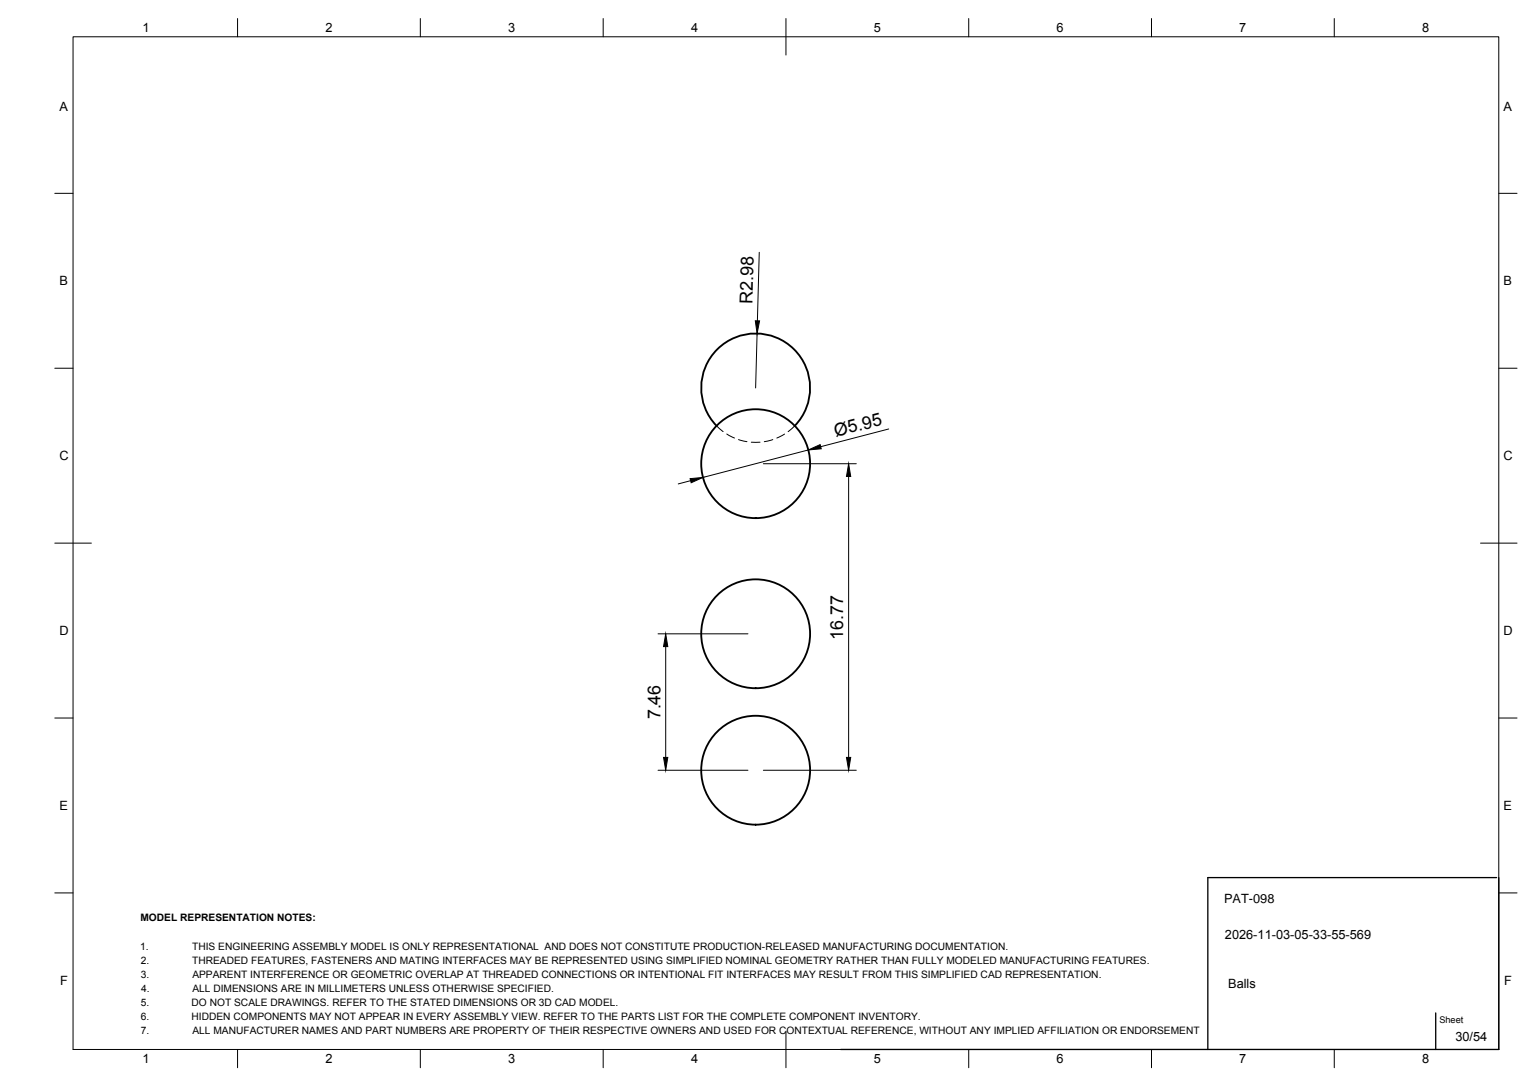
ISO-10303-21;
HEADER;
/* Generated by software containing ST-Developer
 * from STEP Tools, Inc. (www.steptools.com) 
 */

FILE_DESCRIPTION(
/* description */ ('Spring compression tester'),
/* implementation_level */ '2;1');

FILE_NAME(
/* name */ 'Balls.step',
/* time_stamp */ '2026-10-28T03:24:11-07:00',
/* author */ (''),
/* organization */ (''),
/* preprocessor_version */ 'ST-DEVELOPER v20.2',
/* originating_system */ 'Autodesk Translation Framework v15.17.0.0',
/* authorisation */ '');

FILE_SCHEMA (('AUTOMOTIVE_DESIGN { 1 0 10303 214 3 1 1 }'));
ENDSEC;

DATA;
#10=MECHANICAL_DESIGN_GEOMETRIC_PRESENTATION_REPRESENTATION('',(#1129,#1130,#1131,#1132,#1133,#1134,#1135),#43521);
#897=SPHERICAL_SURFACE('',#20034,0.29765);
#898=SPHERICAL_SURFACE('',#20036,0.29765);
#899=SPHERICAL_SURFACE('',#20038,0.29765);
#900=SPHERICAL_SURFACE('',#20040,0.29765);
#901=SPHERICAL_SURFACE('',#20042,0.29765);
#902=SPHERICAL_SURFACE('',#20044,0.29765);
#903=SPHERICAL_SURFACE('',#20046,0.29765);
#1009=SHAPE_REPRESENTATION_RELATIONSHIP('SRR','None',#43822,#1069);
#1069=ADVANCED_BREP_SHAPE_REPRESENTATION('',(#1203,#1204,#1205,#1206,#1207,
#1208,#1209),#43482);
#1129=STYLED_ITEM('',(#44202),#1203);
#1130=STYLED_ITEM('',(#44202),#1204);
#1131=STYLED_ITEM('',(#44202),#1205);
#1132=STYLED_ITEM('',(#44202),#1206);
#1133=STYLED_ITEM('',(#44202),#1207);
#1134=STYLED_ITEM('',(#44202),#1208);
#1135=STYLED_ITEM('',(#44202),#1209);
#1203=MANIFOLD_SOLID_BREP('Body1',#18567);
#1204=MANIFOLD_SOLID_BREP('Body2',#18568);
#1205=MANIFOLD_SOLID_BREP('Body3',#18569);
#1206=MANIFOLD_SOLID_BREP('Body4',#18570);
#1207=MANIFOLD_SOLID_BREP('Body5',#18571);
#1208=MANIFOLD_SOLID_BREP('Body6',#18572);
#1209=MANIFOLD_SOLID_BREP('Body7',#18573);
#2612=FACE_OUTER_BOUND('',#3866,.T.);
#2613=FACE_OUTER_BOUND('',#3867,.T.);
#2614=FACE_OUTER_BOUND('',#3868,.T.);
#2615=FACE_OUTER_BOUND('',#3869,.T.);
#2616=FACE_OUTER_BOUND('',#3870,.T.);
#2617=FACE_OUTER_BOUND('',#3871,.T.);
#2618=FACE_OUTER_BOUND('',#3872,.T.);
#3866=EDGE_LOOP('',(#14185,#14186));
#3867=EDGE_LOOP('',(#14187,#14188));
#3868=EDGE_LOOP('',(#14189,#14190));
#3869=EDGE_LOOP('',(#14191,#14192));
#3870=EDGE_LOOP('',(#14193,#14194));
#3871=EDGE_LOOP('',(#14195,#14196));
#3872=EDGE_LOOP('',(#14197,#14198));
#7749=CIRCLE('',#20035,0.29765);
#7750=CIRCLE('',#20037,0.29765);
#7751=CIRCLE('',#20039,0.29765);
#7752=CIRCLE('',#20041,0.29765);
#7753=CIRCLE('',#20043,0.29765);
#7754=CIRCLE('',#20045,0.29765);
#7755=CIRCLE('',#20047,0.29765);
#8789=VERTEX_POINT('',#28561);
#8790=VERTEX_POINT('',#28562);
#8791=VERTEX_POINT('',#28565);
#8792=VERTEX_POINT('',#28566);
#8793=VERTEX_POINT('',#28569);
#8794=VERTEX_POINT('',#28570);
#8795=VERTEX_POINT('',#28573);
#8796=VERTEX_POINT('',#28574);
#8797=VERTEX_POINT('',#28577);
#8798=VERTEX_POINT('',#28578);
#8799=VERTEX_POINT('',#28581);
#8800=VERTEX_POINT('',#28582);
#8801=VERTEX_POINT('',#28585);
#8802=VERTEX_POINT('',#28586);
#10757=EDGE_CURVE('',#8789,#8790,#7749,.T.);
#10758=EDGE_CURVE('',#8791,#8792,#7750,.T.);
#10759=EDGE_CURVE('',#8793,#8794,#7751,.T.);
#10760=EDGE_CURVE('',#8795,#8796,#7752,.T.);
#10761=EDGE_CURVE('',#8797,#8798,#7753,.T.);
#10762=EDGE_CURVE('',#8799,#8800,#7754,.T.);
#10763=EDGE_CURVE('',#8801,#8802,#7755,.T.);
#14185=ORIENTED_EDGE('',*,*,#10757,.T.);
#14186=ORIENTED_EDGE('',*,*,#10757,.F.);
#14187=ORIENTED_EDGE('',*,*,#10758,.T.);
#14188=ORIENTED_EDGE('',*,*,#10758,.F.);
#14189=ORIENTED_EDGE('',*,*,#10759,.T.);
#14190=ORIENTED_EDGE('',*,*,#10759,.F.);
#14191=ORIENTED_EDGE('',*,*,#10760,.T.);
#14192=ORIENTED_EDGE('',*,*,#10760,.F.);
#14193=ORIENTED_EDGE('',*,*,#10761,.T.);
#14194=ORIENTED_EDGE('',*,*,#10761,.F.);
#14195=ORIENTED_EDGE('',*,*,#10762,.T.);
#14196=ORIENTED_EDGE('',*,*,#10762,.F.);
#14197=ORIENTED_EDGE('',*,*,#10763,.T.);
#14198=ORIENTED_EDGE('',*,*,#10763,.F.);
#17936=ADVANCED_FACE('',(#2612),#897,.T.);
#17937=ADVANCED_FACE('',(#2613),#898,.T.);
#17938=ADVANCED_FACE('',(#2614),#899,.T.);
#17939=ADVANCED_FACE('',(#2615),#900,.T.);
#17940=ADVANCED_FACE('',(#2616),#901,.T.);
#17941=ADVANCED_FACE('',(#2617),#902,.T.);
#17942=ADVANCED_FACE('',(#2618),#903,.T.);
#18567=CLOSED_SHELL('',(#17936));
#18568=CLOSED_SHELL('',(#17937));
#18569=CLOSED_SHELL('',(#17938));
#18570=CLOSED_SHELL('',(#17939));
#18571=CLOSED_SHELL('',(#17940));
#18572=CLOSED_SHELL('',(#17941));
#18573=CLOSED_SHELL('',(#17942));
#20033=AXIS2_PLACEMENT_3D('',#28559,#23399,#23400);
#20034=AXIS2_PLACEMENT_3D('',#28560,#23401,#23402);
#20035=AXIS2_PLACEMENT_3D('',#28563,#23403,#23404);
#20036=AXIS2_PLACEMENT_3D('',#28564,#23405,#23406);
#20037=AXIS2_PLACEMENT_3D('',#28567,#23407,#23408);
#20038=AXIS2_PLACEMENT_3D('',#28568,#23409,#23410);
#20039=AXIS2_PLACEMENT_3D('',#28571,#23411,#23412);
#20040=AXIS2_PLACEMENT_3D('',#28572,#23413,#23414);
#20041=AXIS2_PLACEMENT_3D('',#28575,#23415,#23416);
#20042=AXIS2_PLACEMENT_3D('',#28576,#23417,#23418);
#20043=AXIS2_PLACEMENT_3D('',#28579,#23419,#23420);
#20044=AXIS2_PLACEMENT_3D('',#28580,#23421,#23422);
#20045=AXIS2_PLACEMENT_3D('',#28583,#23423,#23424);
#20046=AXIS2_PLACEMENT_3D('',#28584,#23425,#23426);
#20047=AXIS2_PLACEMENT_3D('',#28587,#23427,#23428);
#23399=DIRECTION('axis',(0.,0.,1.));
#23400=DIRECTION('refdir',(1.,0.,0.));
#23401=DIRECTION('center_axis',(0.,0.,1.));
#23402=DIRECTION('ref_axis',(1.,0.,0.));
#23403=DIRECTION('center_axis',(1.22464679914735E-16,-1.,0.));
#23404=DIRECTION('ref_axis',(-1.,-1.22464679914735E-16,0.));
#23405=DIRECTION('center_axis',(0.78183148246803,0.,0.623489801858733));
#23406=DIRECTION('ref_axis',(0.623489801858734,0.,-0.78183148246803));
#23407=DIRECTION('center_axis',(7.63554790147315E-17,-1.,-9.57467422477103E-17));
#23408=DIRECTION('ref_axis',(-0.623489801858734,-1.22464679914735E-16,0.78183148246803));
#23409=DIRECTION('center_axis',(0.974927912181824,0.,-0.222520933956314));
#23410=DIRECTION('ref_axis',(-0.222520933956314,0.,-0.974927912181824));
#23411=DIRECTION('center_axis',(-2.7250954951288E-17,-1.,-1.19394234705288E-16));
#23412=DIRECTION('ref_axis',(0.222520933956314,-1.22464679914735E-16,0.974927912181824));
#23413=DIRECTION('center_axis',(0.433883739117558,0.,-0.900968867902419));
#23414=DIRECTION('ref_axis',(-0.900968867902419,0.,-0.433883739117558));
#23415=DIRECTION('center_axis',(-1.10336864020811E-16,-1.,-5.31354332312403E-17));
#23416=DIRECTION('ref_axis',(0.900968867902419,-1.22464679914735E-16,0.433883739117558));
#23417=DIRECTION('center_axis',(-0.433883739117558,0.,-0.900968867902419));
#23418=DIRECTION('ref_axis',(-0.900968867902419,0.,0.433883739117558));
#23419=DIRECTION('center_axis',(-1.10336864020811E-16,-1.,5.31354332312403E-17));
#23420=DIRECTION('ref_axis',(0.900968867902419,-1.22464679914735E-16,-0.433883739117558));
#23421=DIRECTION('center_axis',(-0.974927912181824,0.,-0.222520933956314));
#23422=DIRECTION('ref_axis',(-0.222520933956315,0.,0.974927912181824));
#23423=DIRECTION('center_axis',(-2.7250954951288E-17,-1.,1.19394234705288E-16));
#23424=DIRECTION('ref_axis',(0.222520933956315,-1.22464679914735E-16,-0.974927912181824));
#23425=DIRECTION('center_axis',(-0.78183148246803,0.,0.623489801858734));
#23426=DIRECTION('ref_axis',(0.623489801858733,0.,0.78183148246803));
#23427=DIRECTION('center_axis',(7.63554790147315E-17,-1.,9.57467422477103E-17));
#23428=DIRECTION('ref_axis',(-0.623489801858733,-1.22464679914735E-16,-0.78183148246803));
#28559=CARTESIAN_POINT('',(0.,0.,0.));
#28560=CARTESIAN_POINT('Origin',(1.1,0.,0.));
#28561=CARTESIAN_POINT('',(1.1,-2.23201749654651E-33,0.29765));
#28562=CARTESIAN_POINT('',(1.1,-2.23201749654651E-33,-0.29765));
#28563=CARTESIAN_POINT('Origin',(1.1,0.,0.));
#28564=CARTESIAN_POINT('Origin',(0.685838782044607,0.,-0.860014630714833));
#28565=CARTESIAN_POINT('',(0.918550922801216,-5.31350540756609E-33,-0.674432891191581));
#28566=CARTESIAN_POINT('',(0.453126641287998,8.49470414473068E-34,-1.04559637023808));
#28567=CARTESIAN_POINT('Origin',(0.685838782044607,0.,-0.860014630714833));
#28568=CARTESIAN_POINT('Origin',(-0.244773027351946,0.,-1.07242070340001));
#28569=CARTESIAN_POINT('',(0.0454142657089739,-2.23201749654651E-33,-1.1386540593921));
#28570=CARTESIAN_POINT('',(-0.534960320412865,-2.23201749654651E-33,-1.00618734740791));
#28571=CARTESIAN_POINT('Origin',(-0.244773027351946,0.,-1.07242070340001));
#28572=CARTESIAN_POINT('Origin',(-0.991065754692661,0.,-0.477272113029314));
#28573=CARTESIAN_POINT('',(-0.86192025974432,8.49470414473067E-34,-0.745445496560469));
#28574=CARTESIAN_POINT('',(-1.120211249641,-5.31350540756609E-33,-0.209098729498159));
#28575=CARTESIAN_POINT('Origin',(-0.991065754692661,0.,-0.477272113029314));
#28576=CARTESIAN_POINT('Origin',(-0.991065754692661,0.,0.477272113029314));
#28577=CARTESIAN_POINT('',(-1.120211249641,-2.23201749654651E-33,0.209098729498159));
#28578=CARTESIAN_POINT('',(-0.86192025974432,-2.23201749654651E-33,0.745445496560469));
#28579=CARTESIAN_POINT('Origin',(-0.991065754692661,0.,0.477272113029314));
#28580=CARTESIAN_POINT('Origin',(-0.244773027351946,0.,1.07242070340001));
#28581=CARTESIAN_POINT('',(-0.534960320412866,-2.23201749654651E-33,1.00618734740791));
#28582=CARTESIAN_POINT('',(0.0454142657089737,-2.23201749654651E-33,1.1386540593921));
#28583=CARTESIAN_POINT('Origin',(-0.244773027351946,0.,1.07242070340001));
#28584=CARTESIAN_POINT('Origin',(0.685838782044607,0.,0.860014630714833));
#28585=CARTESIAN_POINT('',(0.453126641287998,-2.23201749654651E-33,1.04559637023808));
#28586=CARTESIAN_POINT('',(0.918550922801216,-2.23201749654651E-33,0.674432891191581));
#28587=CARTESIAN_POINT('Origin',(0.685838782044607,0.,0.860014630714833));
#43414=UNCERTAINTY_MEASURE_WITH_UNIT(LENGTH_MEASURE(0.001),#43522,
'DISTANCE_ACCURACY_VALUE',
'Maximum model space distance between geometric entities at asserted c
onnectivities');
#43453=UNCERTAINTY_MEASURE_WITH_UNIT(LENGTH_MEASURE(0.001),#43522,
'DISTANCE_ACCURACY_VALUE',
'Maximum model space distance between geometric entities at asserted c
onnectivities');
#43482=(
GEOMETRIC_REPRESENTATION_CONTEXT(3)
GLOBAL_UNCERTAINTY_ASSIGNED_CONTEXT((#43414))
GLOBAL_UNIT_ASSIGNED_CONTEXT((#43522,#43524,#43525))
REPRESENTATION_CONTEXT('','3D')
);
#43521=(
GEOMETRIC_REPRESENTATION_CONTEXT(3)
GLOBAL_UNCERTAINTY_ASSIGNED_CONTEXT((#43453))
GLOBAL_UNIT_ASSIGNED_CONTEXT((#43522,#43524,#43525))
REPRESENTATION_CONTEXT('','3D')
);
#43522=(
LENGTH_UNIT()
NAMED_UNIT(*)
SI_UNIT(.CENTI.,.METRE.)
);
#43524=(
NAMED_UNIT(*)
PLANE_ANGLE_UNIT()
SI_UNIT($,.RADIAN.)
);
#43525=(
NAMED_UNIT(*)
SI_UNIT($,.STERADIAN.)
SOLID_ANGLE_UNIT()
);
#43554=SHAPE_DEFINITION_REPRESENTATION(#43621,#43822);
#43621=PRODUCT_DEFINITION_SHAPE('',$,#43890);
#43822=SHAPE_REPRESENTATION('',(#20033),#43482);
#43861=PRODUCT_DEFINITION_CONTEXT('part definition',#44064,'design');
#43890=PRODUCT_DEFINITION('Balls','Balls',#43957,#43861);
#43957=PRODUCT_DEFINITION_FORMATION('',$,#44094);
#44064=APPLICATION_CONTEXT(
'Core Data for Automotive Mechanical Design Process');
#44065=PRODUCT_CONTEXT('part definition',#44064,'mechanical');
#44094=PRODUCT('Balls','Balls','Balls',(#44065));
#44196=COLOUR_RGB('Grey',0.48,0.52,0.57);
#44197=FILL_AREA_STYLE_COLOUR('',#44196);
#44198=FILL_AREA_STYLE('',(#44197));
#44199=SURFACE_STYLE_FILL_AREA(#44198);
#44200=SURFACE_SIDE_STYLE('',(#44199));
#44201=SURFACE_STYLE_USAGE(.BOTH.,#44200);
#44202=PRESENTATION_STYLE_ASSIGNMENT((#44201));
ENDSEC;
END-ISO-10303-21;
